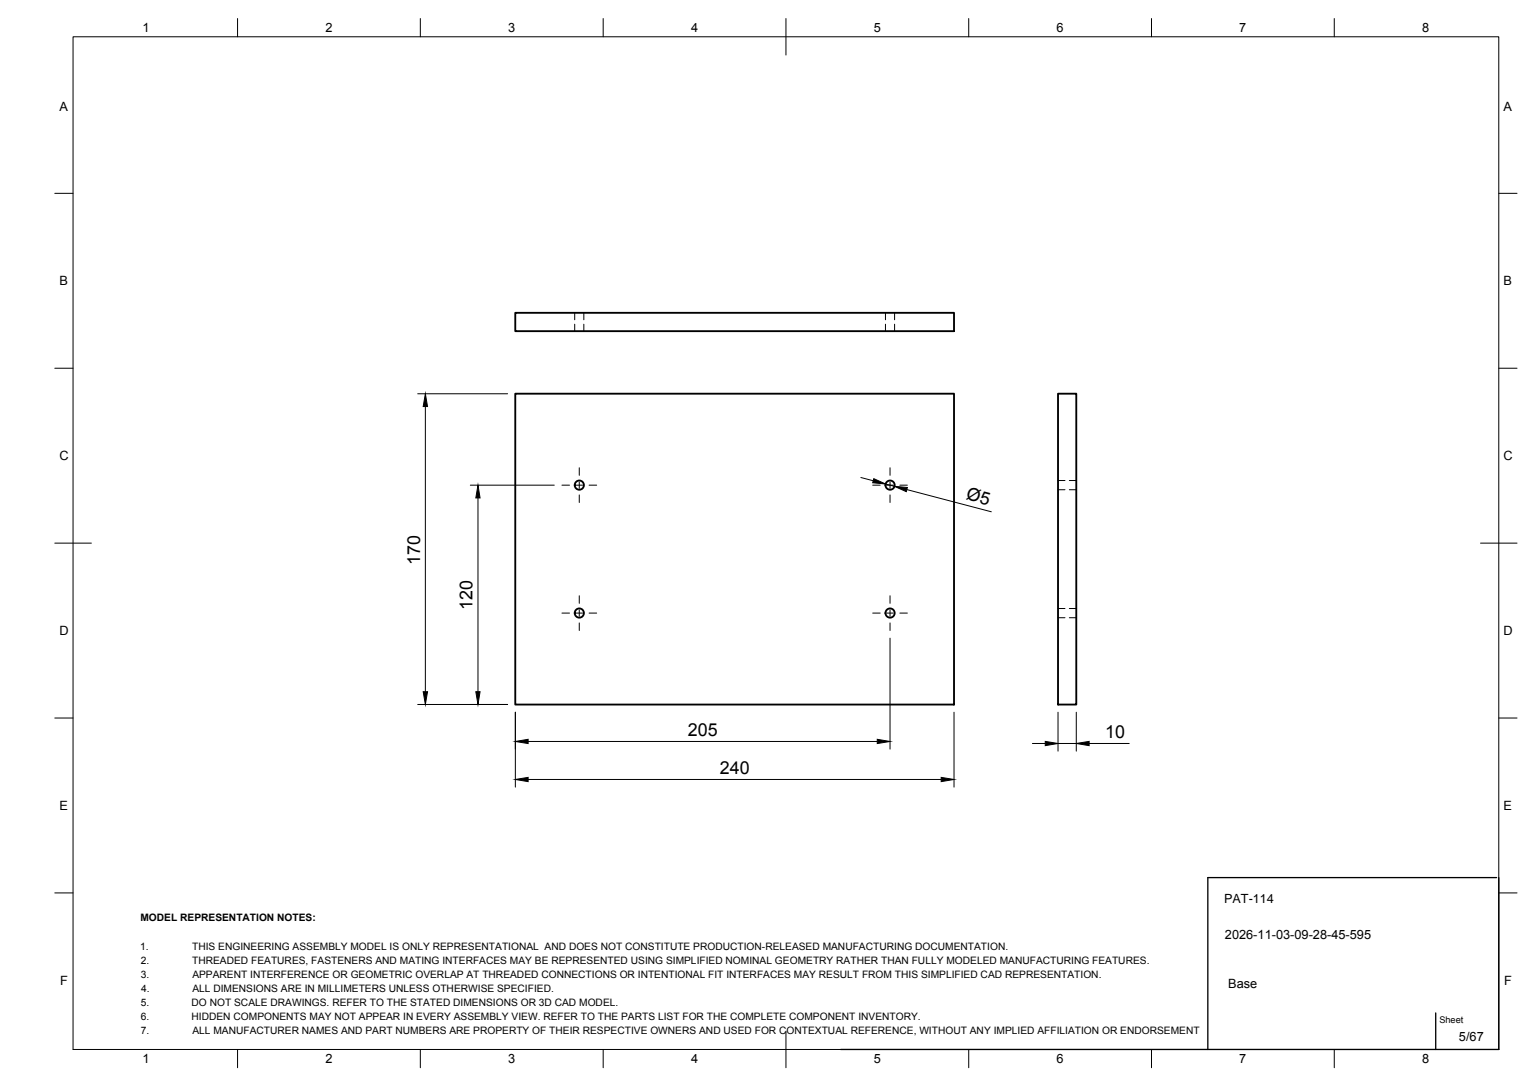
ISO-10303-21;
HEADER;
/* Generated by software containing ST-Developer
 * from STEP Tools, Inc. (www.steptools.com) 
 */

FILE_DESCRIPTION(
/* description */ ('Two-stage gear reducer in split housing'),
/* implementation_level */ '2;1');

FILE_NAME(
/* name */ 'Base.step',
/* time_stamp */ '2026-10-28T03:22:31-07:00',
/* author */ (''),
/* organization */ (''),
/* preprocessor_version */ 'ST-DEVELOPER v20.2',
/* originating_system */ 'Autodesk Translation Framework v15.17.0.0',
/* authorisation */ '');

FILE_SCHEMA (('AUTOMOTIVE_DESIGN { 1 0 10303 214 3 1 1 }'));
ENDSEC;

DATA;
#10=MECHANICAL_DESIGN_GEOMETRIC_PRESENTATION_REPRESENTATION('',(#1234),#73366);
#1122=SHAPE_REPRESENTATION_RELATIONSHIP('SRR','None',#73609,#1178);
#1178=ADVANCED_BREP_SHAPE_REPRESENTATION('',(#1305),#73305);
#1234=STYLED_ITEM('',(#73967),#1305);
#1305=MANIFOLD_SOLID_BREP('Body1',#16122);
#1374=FACE_BOUND('',#2924,.T.);
#1375=FACE_BOUND('',#2925,.T.);
#1376=FACE_BOUND('',#2926,.T.);
#1377=FACE_BOUND('',#2927,.T.);
#1378=FACE_BOUND('',#2929,.T.);
#1379=FACE_BOUND('',#2930,.T.);
#1380=FACE_BOUND('',#2931,.T.);
#1381=FACE_BOUND('',#2932,.T.);
#1602=PLANE('',#16827);
#1603=PLANE('',#16828);
#1604=PLANE('',#16829);
#1605=PLANE('',#16830);
#1606=PLANE('',#16831);
#1607=PLANE('',#16832);
#2002=FACE_OUTER_BOUND('',#2915,.T.);
#2003=FACE_OUTER_BOUND('',#2916,.T.);
#2004=FACE_OUTER_BOUND('',#2917,.T.);
#2005=FACE_OUTER_BOUND('',#2918,.T.);
#2006=FACE_OUTER_BOUND('',#2919,.T.);
#2007=FACE_OUTER_BOUND('',#2920,.T.);
#2008=FACE_OUTER_BOUND('',#2921,.T.);
#2009=FACE_OUTER_BOUND('',#2922,.T.);
#2010=FACE_OUTER_BOUND('',#2923,.T.);
#2011=FACE_OUTER_BOUND('',#2928,.T.);
#2915=EDGE_LOOP('',(#10507,#10508,#10509,#10510));
#2916=EDGE_LOOP('',(#10511,#10512,#10513,#10514));
#2917=EDGE_LOOP('',(#10515,#10516,#10517,#10518));
#2918=EDGE_LOOP('',(#10519,#10520,#10521,#10522));
#2919=EDGE_LOOP('',(#10523,#10524,#10525,#10526));
#2920=EDGE_LOOP('',(#10527,#10528,#10529,#10530));
#2921=EDGE_LOOP('',(#10531,#10532,#10533,#10534));
#2922=EDGE_LOOP('',(#10535,#10536,#10537,#10538));
#2923=EDGE_LOOP('',(#10539,#10540,#10541,#10542));
#2924=EDGE_LOOP('',(#10543));
#2925=EDGE_LOOP('',(#10544));
#2926=EDGE_LOOP('',(#10545));
#2927=EDGE_LOOP('',(#10546));
#2928=EDGE_LOOP('',(#10547,#10548,#10549,#10550));
#2929=EDGE_LOOP('',(#10551));
#2930=EDGE_LOOP('',(#10552));
#2931=EDGE_LOOP('',(#10553));
#2932=EDGE_LOOP('',(#10554));
#4056=LINE('',#22781,#5080);
#4057=LINE('',#22787,#5081);
#4058=LINE('',#22793,#5082);
#4059=LINE('',#22799,#5083);
#4060=LINE('',#22804,#5084);
#4061=LINE('',#22806,#5085);
#4062=LINE('',#22808,#5086);
#4063=LINE('',#22809,#5087);
#4064=LINE('',#22812,#5088);
#4065=LINE('',#22814,#5089);
#4066=LINE('',#22815,#5090);
#4067=LINE('',#22818,#5091);
#4068=LINE('',#22820,#5092);
#4069=LINE('',#22821,#5093);
#4070=LINE('',#22823,#5094);
#4071=LINE('',#22824,#5095);
#5080=VECTOR('',#18468,0.25);
#5081=VECTOR('',#18475,0.25);
#5082=VECTOR('',#18482,0.25);
#5083=VECTOR('',#18489,0.25);
#5084=VECTOR('',#18494,1.);
#5085=VECTOR('',#18495,1.);
#5086=VECTOR('',#18496,1.);
#5087=VECTOR('',#18497,1.);
#5088=VECTOR('',#18500,1.);
#5089=VECTOR('',#18501,1.);
#5090=VECTOR('',#18502,1.);
#5091=VECTOR('',#18505,1.);
#5092=VECTOR('',#18506,1.);
#5093=VECTOR('',#18507,1.);
#5094=VECTOR('',#18510,1.);
#5095=VECTOR('',#18511,1.);
#6104=CIRCLE('',#16816,0.25);
#6105=CIRCLE('',#16817,0.25);
#6106=CIRCLE('',#16819,0.25);
#6107=CIRCLE('',#16820,0.25);
#6108=CIRCLE('',#16822,0.25);
#6109=CIRCLE('',#16823,0.25);
#6110=CIRCLE('',#16825,0.25);
#6111=CIRCLE('',#16826,0.25);
#6824=VERTEX_POINT('',#22778);
#6825=VERTEX_POINT('',#22780);
#6826=VERTEX_POINT('',#22784);
#6827=VERTEX_POINT('',#22786);
#6828=VERTEX_POINT('',#22790);
#6829=VERTEX_POINT('',#22792);
#6830=VERTEX_POINT('',#22796);
#6831=VERTEX_POINT('',#22798);
#6832=VERTEX_POINT('',#22802);
#6833=VERTEX_POINT('',#22803);
#6834=VERTEX_POINT('',#22805);
#6835=VERTEX_POINT('',#22807);
#6836=VERTEX_POINT('',#22811);
#6837=VERTEX_POINT('',#22813);
#6838=VERTEX_POINT('',#22817);
#6839=VERTEX_POINT('',#22819);
#8307=EDGE_CURVE('',#6824,#6824,#6104,.T.);
#8308=EDGE_CURVE('',#6824,#6825,#4056,.T.);
#8309=EDGE_CURVE('',#6825,#6825,#6105,.T.);
#8310=EDGE_CURVE('',#6826,#6826,#6106,.T.);
#8311=EDGE_CURVE('',#6826,#6827,#4057,.T.);
#8312=EDGE_CURVE('',#6827,#6827,#6107,.T.);
#8313=EDGE_CURVE('',#6828,#6828,#6108,.T.);
#8314=EDGE_CURVE('',#6828,#6829,#4058,.T.);
#8315=EDGE_CURVE('',#6829,#6829,#6109,.T.);
#8316=EDGE_CURVE('',#6830,#6830,#6110,.T.);
#8317=EDGE_CURVE('',#6830,#6831,#4059,.T.);
#8318=EDGE_CURVE('',#6831,#6831,#6111,.T.);
#8319=EDGE_CURVE('',#6832,#6833,#4060,.T.);
#8320=EDGE_CURVE('',#6833,#6834,#4061,.T.);
#8321=EDGE_CURVE('',#6835,#6834,#4062,.T.);
#8322=EDGE_CURVE('',#6832,#6835,#4063,.T.);
#8323=EDGE_CURVE('',#6836,#6832,#4064,.T.);
#8324=EDGE_CURVE('',#6837,#6835,#4065,.T.);
#8325=EDGE_CURVE('',#6836,#6837,#4066,.T.);
#8326=EDGE_CURVE('',#6838,#6836,#4067,.T.);
#8327=EDGE_CURVE('',#6839,#6837,#4068,.T.);
#8328=EDGE_CURVE('',#6838,#6839,#4069,.T.);
#8329=EDGE_CURVE('',#6833,#6838,#4070,.T.);
#8330=EDGE_CURVE('',#6834,#6839,#4071,.T.);
#10507=ORIENTED_EDGE('',*,*,#8307,.F.);
#10508=ORIENTED_EDGE('',*,*,#8308,.T.);
#10509=ORIENTED_EDGE('',*,*,#8309,.F.);
#10510=ORIENTED_EDGE('',*,*,#8308,.F.);
#10511=ORIENTED_EDGE('',*,*,#8310,.F.);
#10512=ORIENTED_EDGE('',*,*,#8311,.T.);
#10513=ORIENTED_EDGE('',*,*,#8312,.F.);
#10514=ORIENTED_EDGE('',*,*,#8311,.F.);
#10515=ORIENTED_EDGE('',*,*,#8313,.F.);
#10516=ORIENTED_EDGE('',*,*,#8314,.T.);
#10517=ORIENTED_EDGE('',*,*,#8315,.F.);
#10518=ORIENTED_EDGE('',*,*,#8314,.F.);
#10519=ORIENTED_EDGE('',*,*,#8316,.F.);
#10520=ORIENTED_EDGE('',*,*,#8317,.T.);
#10521=ORIENTED_EDGE('',*,*,#8318,.F.);
#10522=ORIENTED_EDGE('',*,*,#8317,.F.);
#10523=ORIENTED_EDGE('',*,*,#8319,.T.);
#10524=ORIENTED_EDGE('',*,*,#8320,.T.);
#10525=ORIENTED_EDGE('',*,*,#8321,.F.);
#10526=ORIENTED_EDGE('',*,*,#8322,.F.);
#10527=ORIENTED_EDGE('',*,*,#8323,.T.);
#10528=ORIENTED_EDGE('',*,*,#8322,.T.);
#10529=ORIENTED_EDGE('',*,*,#8324,.F.);
#10530=ORIENTED_EDGE('',*,*,#8325,.F.);
#10531=ORIENTED_EDGE('',*,*,#8326,.T.);
#10532=ORIENTED_EDGE('',*,*,#8325,.T.);
#10533=ORIENTED_EDGE('',*,*,#8327,.F.);
#10534=ORIENTED_EDGE('',*,*,#8328,.F.);
#10535=ORIENTED_EDGE('',*,*,#8329,.T.);
#10536=ORIENTED_EDGE('',*,*,#8328,.T.);
#10537=ORIENTED_EDGE('',*,*,#8330,.F.);
#10538=ORIENTED_EDGE('',*,*,#8320,.F.);
#10539=ORIENTED_EDGE('',*,*,#8330,.T.);
#10540=ORIENTED_EDGE('',*,*,#8327,.T.);
#10541=ORIENTED_EDGE('',*,*,#8324,.T.);
#10542=ORIENTED_EDGE('',*,*,#8321,.T.);
#10543=ORIENTED_EDGE('',*,*,#8309,.T.);
#10544=ORIENTED_EDGE('',*,*,#8312,.T.);
#10545=ORIENTED_EDGE('',*,*,#8315,.T.);
#10546=ORIENTED_EDGE('',*,*,#8318,.T.);
#10547=ORIENTED_EDGE('',*,*,#8329,.F.);
#10548=ORIENTED_EDGE('',*,*,#8319,.F.);
#10549=ORIENTED_EDGE('',*,*,#8323,.F.);
#10550=ORIENTED_EDGE('',*,*,#8326,.F.);
#10551=ORIENTED_EDGE('',*,*,#8307,.T.);
#10552=ORIENTED_EDGE('',*,*,#8310,.T.);
#10553=ORIENTED_EDGE('',*,*,#8313,.T.);
#10554=ORIENTED_EDGE('',*,*,#8316,.T.);
#14907=CYLINDRICAL_SURFACE('',#16815,0.25);
#14908=CYLINDRICAL_SURFACE('',#16818,0.25);
#14909=CYLINDRICAL_SURFACE('',#16821,0.25);
#14910=CYLINDRICAL_SURFACE('',#16824,0.25);
#15209=ADVANCED_FACE('',(#2002),#14907,.F.);
#15210=ADVANCED_FACE('',(#2003),#14908,.F.);
#15211=ADVANCED_FACE('',(#2004),#14909,.F.);
#15212=ADVANCED_FACE('',(#2005),#14910,.F.);
#15213=ADVANCED_FACE('',(#2006),#1602,.T.);
#15214=ADVANCED_FACE('',(#2007),#1603,.T.);
#15215=ADVANCED_FACE('',(#2008),#1604,.T.);
#15216=ADVANCED_FACE('',(#2009),#1605,.T.);
#15217=ADVANCED_FACE('',(#2010,#1374,#1375,#1376,#1377),#1606,.T.);
#15218=ADVANCED_FACE('',(#2011,#1378,#1379,#1380,#1381),#1607,.F.);
#16122=CLOSED_SHELL('',(#15209,#15210,#15211,#15212,#15213,#15214,#15215,
#15216,#15217,#15218));
#16814=AXIS2_PLACEMENT_3D('',#22776,#18462,#18463);
#16815=AXIS2_PLACEMENT_3D('',#22777,#18464,#18465);
#16816=AXIS2_PLACEMENT_3D('',#22779,#18466,#18467);
#16817=AXIS2_PLACEMENT_3D('',#22782,#18469,#18470);
#16818=AXIS2_PLACEMENT_3D('',#22783,#18471,#18472);
#16819=AXIS2_PLACEMENT_3D('',#22785,#18473,#18474);
#16820=AXIS2_PLACEMENT_3D('',#22788,#18476,#18477);
#16821=AXIS2_PLACEMENT_3D('',#22789,#18478,#18479);
#16822=AXIS2_PLACEMENT_3D('',#22791,#18480,#18481);
#16823=AXIS2_PLACEMENT_3D('',#22794,#18483,#18484);
#16824=AXIS2_PLACEMENT_3D('',#22795,#18485,#18486);
#16825=AXIS2_PLACEMENT_3D('',#22797,#18487,#18488);
#16826=AXIS2_PLACEMENT_3D('',#22800,#18490,#18491);
#16827=AXIS2_PLACEMENT_3D('',#22801,#18492,#18493);
#16828=AXIS2_PLACEMENT_3D('',#22810,#18498,#18499);
#16829=AXIS2_PLACEMENT_3D('',#22816,#18503,#18504);
#16830=AXIS2_PLACEMENT_3D('',#22822,#18508,#18509);
#16831=AXIS2_PLACEMENT_3D('',#22825,#18512,#18513);
#16832=AXIS2_PLACEMENT_3D('',#22826,#18514,#18515);
#18462=DIRECTION('axis',(0.,0.,1.));
#18463=DIRECTION('refdir',(1.,0.,0.));
#18464=DIRECTION('center_axis',(0.,0.,1.));
#18465=DIRECTION('ref_axis',(1.,0.,0.));
#18466=DIRECTION('center_axis',(0.,0.,1.));
#18467=DIRECTION('ref_axis',(1.,0.,0.));
#18468=DIRECTION('',(0.,0.,1.));
#18469=DIRECTION('center_axis',(0.,0.,-1.));
#18470=DIRECTION('ref_axis',(1.,0.,0.));
#18471=DIRECTION('center_axis',(0.,0.,1.));
#18472=DIRECTION('ref_axis',(1.,0.,0.));
#18473=DIRECTION('center_axis',(0.,0.,1.));
#18474=DIRECTION('ref_axis',(1.,0.,0.));
#18475=DIRECTION('',(0.,0.,1.));
#18476=DIRECTION('center_axis',(0.,0.,-1.));
#18477=DIRECTION('ref_axis',(1.,0.,0.));
#18478=DIRECTION('center_axis',(0.,0.,1.));
#18479=DIRECTION('ref_axis',(1.,0.,0.));
#18480=DIRECTION('center_axis',(0.,0.,1.));
#18481=DIRECTION('ref_axis',(1.,0.,0.));
#18482=DIRECTION('',(0.,0.,1.));
#18483=DIRECTION('center_axis',(0.,0.,-1.));
#18484=DIRECTION('ref_axis',(1.,0.,0.));
#18485=DIRECTION('center_axis',(0.,0.,1.));
#18486=DIRECTION('ref_axis',(1.,0.,0.));
#18487=DIRECTION('center_axis',(0.,0.,1.));
#18488=DIRECTION('ref_axis',(1.,0.,0.));
#18489=DIRECTION('',(0.,0.,1.));
#18490=DIRECTION('center_axis',(0.,0.,-1.));
#18491=DIRECTION('ref_axis',(1.,0.,0.));
#18492=DIRECTION('center_axis',(0.,1.,0.));
#18493=DIRECTION('ref_axis',(-1.,0.,0.));
#18494=DIRECTION('',(-1.,0.,0.));
#18495=DIRECTION('',(0.,0.,1.));
#18496=DIRECTION('',(-1.,0.,0.));
#18497=DIRECTION('',(0.,0.,1.));
#18498=DIRECTION('center_axis',(1.,0.,0.));
#18499=DIRECTION('ref_axis',(0.,1.,0.));
#18500=DIRECTION('',(0.,1.,0.));
#18501=DIRECTION('',(0.,1.,0.));
#18502=DIRECTION('',(0.,0.,1.));
#18503=DIRECTION('center_axis',(0.,-1.,0.));
#18504=DIRECTION('ref_axis',(1.,0.,0.));
#18505=DIRECTION('',(1.,0.,0.));
#18506=DIRECTION('',(1.,0.,0.));
#18507=DIRECTION('',(0.,0.,1.));
#18508=DIRECTION('center_axis',(-1.,0.,0.));
#18509=DIRECTION('ref_axis',(0.,-1.,0.));
#18510=DIRECTION('',(0.,-1.,0.));
#18511=DIRECTION('',(0.,-1.,0.));
#18512=DIRECTION('center_axis',(0.,0.,1.));
#18513=DIRECTION('ref_axis',(1.,0.,0.));
#18514=DIRECTION('center_axis',(0.,0.,1.));
#18515=DIRECTION('ref_axis',(1.,0.,0.));
#22776=CARTESIAN_POINT('',(0.,0.,0.));
#22777=CARTESIAN_POINT('Origin',(15.,-3.5,-0.1));
#22778=CARTESIAN_POINT('',(14.75,-3.5,0.));
#22779=CARTESIAN_POINT('Origin',(15.,-3.5,0.));
#22780=CARTESIAN_POINT('',(14.75,-3.5,1.));
#22781=CARTESIAN_POINT('',(14.75,-3.5,-0.1));
#22782=CARTESIAN_POINT('Origin',(15.,-3.5,1.));
#22783=CARTESIAN_POINT('Origin',(-2.,3.5,-0.1));
#22784=CARTESIAN_POINT('',(-2.25,3.5,0.));
#22785=CARTESIAN_POINT('Origin',(-2.,3.5,0.));
#22786=CARTESIAN_POINT('',(-2.25,3.5,1.));
#22787=CARTESIAN_POINT('',(-2.25,3.5,-0.1));
#22788=CARTESIAN_POINT('Origin',(-2.,3.5,1.));
#22789=CARTESIAN_POINT('Origin',(-2.,-3.5,-0.1));
#22790=CARTESIAN_POINT('',(-2.25,-3.5,0.));
#22791=CARTESIAN_POINT('Origin',(-2.,-3.5,0.));
#22792=CARTESIAN_POINT('',(-2.25,-3.5,1.));
#22793=CARTESIAN_POINT('',(-2.25,-3.5,-0.1));
#22794=CARTESIAN_POINT('Origin',(-2.,-3.5,1.));
#22795=CARTESIAN_POINT('Origin',(15.,3.5,-0.1));
#22796=CARTESIAN_POINT('',(14.75,3.5,0.));
#22797=CARTESIAN_POINT('Origin',(15.,3.5,0.));
#22798=CARTESIAN_POINT('',(14.75,3.5,1.));
#22799=CARTESIAN_POINT('',(14.75,3.5,-0.1));
#22800=CARTESIAN_POINT('Origin',(15.,3.5,1.));
#22801=CARTESIAN_POINT('Origin',(18.5,8.5,0.));
#22802=CARTESIAN_POINT('',(18.5,8.5,0.));
#22803=CARTESIAN_POINT('',(-5.5,8.5,0.));
#22804=CARTESIAN_POINT('',(18.5,8.5,0.));
#22805=CARTESIAN_POINT('',(-5.5,8.5,1.));
#22806=CARTESIAN_POINT('',(-5.5,8.5,0.));
#22807=CARTESIAN_POINT('',(18.5,8.5,1.));
#22808=CARTESIAN_POINT('',(18.5,8.5,1.));
#22809=CARTESIAN_POINT('',(18.5,8.5,0.));
#22810=CARTESIAN_POINT('Origin',(18.5,-8.5,0.));
#22811=CARTESIAN_POINT('',(18.5,-8.5,0.));
#22812=CARTESIAN_POINT('',(18.5,-8.5,0.));
#22813=CARTESIAN_POINT('',(18.5,-8.5,1.));
#22814=CARTESIAN_POINT('',(18.5,-8.5,1.));
#22815=CARTESIAN_POINT('',(18.5,-8.5,0.));
#22816=CARTESIAN_POINT('Origin',(-5.5,-8.5,0.));
#22817=CARTESIAN_POINT('',(-5.5,-8.5,0.));
#22818=CARTESIAN_POINT('',(-5.5,-8.5,0.));
#22819=CARTESIAN_POINT('',(-5.5,-8.5,1.));
#22820=CARTESIAN_POINT('',(-5.5,-8.5,1.));
#22821=CARTESIAN_POINT('',(-5.5,-8.5,0.));
#22822=CARTESIAN_POINT('Origin',(-5.5,8.5,0.));
#22823=CARTESIAN_POINT('',(-5.5,8.5,0.));
#22824=CARTESIAN_POINT('',(-5.5,8.5,1.));
#22825=CARTESIAN_POINT('Origin',(6.5,0.,1.));
#22826=CARTESIAN_POINT('Origin',(6.5,0.,0.));
#73241=UNCERTAINTY_MEASURE_WITH_UNIT(LENGTH_MEASURE(0.001),#73367,
'DISTANCE_ACCURACY_VALUE',
'Maximum model space distance between geometric entities at asserted c
onnectivities');
#73302=UNCERTAINTY_MEASURE_WITH_UNIT(LENGTH_MEASURE(0.001),#73367,
'DISTANCE_ACCURACY_VALUE',
'Maximum model space distance between geometric entities at asserted c
onnectivities');
#73305=(
GEOMETRIC_REPRESENTATION_CONTEXT(3)
GLOBAL_UNCERTAINTY_ASSIGNED_CONTEXT((#73241))
GLOBAL_UNIT_ASSIGNED_CONTEXT((#73367,#73369,#73370))
REPRESENTATION_CONTEXT('','3D')
);
#73366=(
GEOMETRIC_REPRESENTATION_CONTEXT(3)
GLOBAL_UNCERTAINTY_ASSIGNED_CONTEXT((#73302))
GLOBAL_UNIT_ASSIGNED_CONTEXT((#73367,#73369,#73370))
REPRESENTATION_CONTEXT('','3D')
);
#73367=(
LENGTH_UNIT()
NAMED_UNIT(*)
SI_UNIT(.CENTI.,.METRE.)
);
#73369=(
NAMED_UNIT(*)
PLANE_ANGLE_UNIT()
SI_UNIT($,.RADIAN.)
);
#73370=(
NAMED_UNIT(*)
SI_UNIT($,.STERADIAN.)
SOLID_ANGLE_UNIT()
);
#73373=SHAPE_DEFINITION_REPRESENTATION(#73436,#73609);
#73436=PRODUCT_DEFINITION_SHAPE('',$,#73673);
#73609=SHAPE_REPRESENTATION('',(#16814),#73305);
#73670=PRODUCT_DEFINITION_CONTEXT('part definition',#73861,'design');
#73673=PRODUCT_DEFINITION('Base','Base',#73736,#73670);
#73736=PRODUCT_DEFINITION_FORMATION('',$,#73865);
#73861=APPLICATION_CONTEXT(
'Core Data for Automotive Mechanical Design Process');
#73862=PRODUCT_CONTEXT('part definition',#73861,'mechanical');
#73865=PRODUCT('Base','Base','Base',(#73862));
#73961=COLOUR_RGB('Dark Blue',0.08,0.2,0.34);
#73962=FILL_AREA_STYLE_COLOUR('',#73961);
#73963=FILL_AREA_STYLE('',(#73962));
#73964=SURFACE_STYLE_FILL_AREA(#73963);
#73965=SURFACE_SIDE_STYLE('',(#73964));
#73966=SURFACE_STYLE_USAGE(.BOTH.,#73965);
#73967=PRESENTATION_STYLE_ASSIGNMENT((#73966));
ENDSEC;
END-ISO-10303-21;
